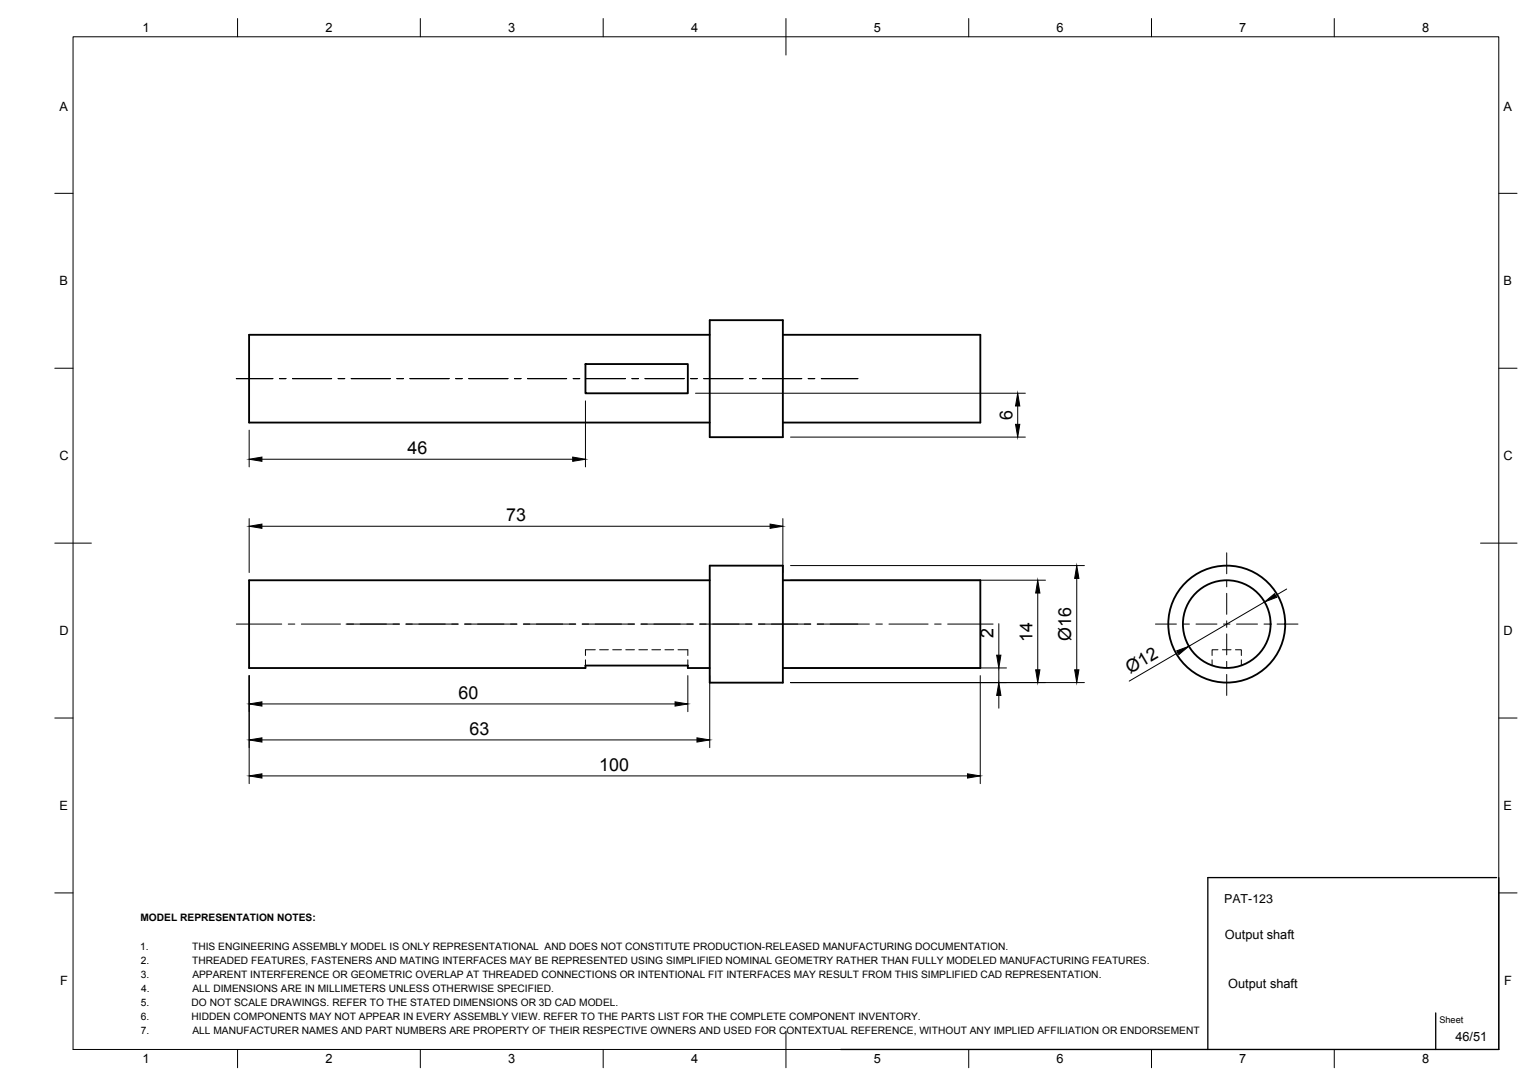
ISO-10303-21;
HEADER;
/* Generated by software containing ST-Developer
 * from STEP Tools, Inc. (www.steptools.com) 
 */

FILE_DESCRIPTION(
/* description */ ('Worm-less right-angle friction wheel drive'),
/* implementation_level */ '2;1');

FILE_NAME(
/* name */ 'Output shaft.step',
/* time_stamp */ '2026-10-28T03:22:36-07:00',
/* author */ (''),
/* organization */ (''),
/* preprocessor_version */ 'ST-DEVELOPER v20.2',
/* originating_system */ 'Autodesk Translation Framework v15.17.0.0',
/* authorisation */ '');

FILE_SCHEMA (('AUTOMOTIVE_DESIGN { 1 0 10303 214 3 1 1 }'));
ENDSEC;

DATA;
#10=MECHANICAL_DESIGN_GEOMETRIC_PRESENTATION_REPRESENTATION('',(#657),#17046);
#556=SHAPE_REPRESENTATION_RELATIONSHIP('SRR','None',#17302,#603);
#603=ADVANCED_BREP_SHAPE_REPRESENTATION('',(#707),#17038);
#657=STYLED_ITEM('',(#17591),#707);
#707=MANIFOLD_SOLID_BREP('Body1',#8216);
#937=FACE_BOUND('',#2304,.T.);
#938=FACE_BOUND('',#2306,.T.);
#939=FACE_BOUND('',#2310,.T.);
#1162=PLANE('',#9644);
#1163=PLANE('',#9645);
#1164=PLANE('',#9647);
#1165=PLANE('',#9648);
#1166=PLANE('',#9649);
#1167=PLANE('',#9651);
#1168=PLANE('',#9654);
#1169=PLANE('',#9662);
#1170=PLANE('',#9663);
#1610=FACE_OUTER_BOUND('',#2298,.T.);
#1611=FACE_OUTER_BOUND('',#2299,.T.);
#1612=FACE_OUTER_BOUND('',#2300,.T.);
#1613=FACE_OUTER_BOUND('',#2301,.T.);
#1614=FACE_OUTER_BOUND('',#2302,.T.);
#1615=FACE_OUTER_BOUND('',#2303,.T.);
#1616=FACE_OUTER_BOUND('',#2305,.T.);
#1617=FACE_OUTER_BOUND('',#2307,.T.);
#1618=FACE_OUTER_BOUND('',#2308,.T.);
#1619=FACE_OUTER_BOUND('',#2309,.T.);
#1620=FACE_OUTER_BOUND('',#2311,.T.);
#1621=FACE_OUTER_BOUND('',#2312,.T.);
#2298=EDGE_LOOP('',(#7254,#7255,#7256,#7257));
#2299=EDGE_LOOP('',(#7258,#7259,#7260,#7261));
#2300=EDGE_LOOP('',(#7262,#7263,#7264,#7265));
#2301=EDGE_LOOP('',(#7266,#7267,#7268,#7269));
#2302=EDGE_LOOP('',(#7270,#7271,#7272,#7273));
#2303=EDGE_LOOP('',(#7274));
#2304=EDGE_LOOP('',(#7275));
#2305=EDGE_LOOP('',(#7276));
#2306=EDGE_LOOP('',(#7277));
#2307=EDGE_LOOP('',(#7278,#7279,#7280,#7281));
#2308=EDGE_LOOP('',(#7282,#7283,#7284,#7285));
#2309=EDGE_LOOP('',(#7286,#7287,#7288,#7289));
#2310=EDGE_LOOP('',(#7290,#7291,#7292,#7293));
#2311=EDGE_LOOP('',(#7294));
#2312=EDGE_LOOP('',(#7295));
#2830=LINE('',#16513,#3370);
#2831=LINE('',#16515,#3371);
#2832=LINE('',#16517,#3372);
#2833=LINE('',#16518,#3373);
#2834=LINE('',#16523,#3374);
#2835=LINE('',#16524,#3375);
#2836=LINE('',#16527,#3376);
#2837=LINE('',#16528,#3377);
#2838=LINE('',#16531,#3378);
#2839=LINE('',#16532,#3379);
#2840=LINE('',#16546,#3380);
#2841=LINE('',#16549,#3381);
#2842=LINE('',#16554,#3382);
#3370=VECTOR('',#12032,1.);
#3371=VECTOR('',#12033,1.);
#3372=VECTOR('',#12034,1.);
#3373=VECTOR('',#12035,1.);
#3374=VECTOR('',#12040,1.);
#3375=VECTOR('',#12041,1.);
#3376=VECTOR('',#12044,1.);
#3377=VECTOR('',#12045,1.);
#3378=VECTOR('',#12048,1.);
#3379=VECTOR('',#12049,1.);
#3380=VECTOR('',#12068,0.8);
#3381=VECTOR('',#12071,0.6);
#3382=VECTOR('',#12078,0.6);
#3832=CIRCLE('',#9646,0.6);
#3833=CIRCLE('',#9650,0.6);
#3834=CIRCLE('',#9652,0.8);
#3835=CIRCLE('',#9653,0.6);
#3836=CIRCLE('',#9655,0.8);
#3837=CIRCLE('',#9656,0.6);
#3838=CIRCLE('',#9659,0.6);
#3839=CIRCLE('',#9661,0.6);
#4445=VERTEX_POINT('',#16511);
#4446=VERTEX_POINT('',#16512);
#4447=VERTEX_POINT('',#16514);
#4448=VERTEX_POINT('',#16516);
#4449=VERTEX_POINT('',#16520);
#4450=VERTEX_POINT('',#16522);
#4451=VERTEX_POINT('',#16526);
#4452=VERTEX_POINT('',#16530);
#4453=VERTEX_POINT('',#16536);
#4454=VERTEX_POINT('',#16538);
#4455=VERTEX_POINT('',#16541);
#4456=VERTEX_POINT('',#16543);
#4457=VERTEX_POINT('',#16548);
#4458=VERTEX_POINT('',#16552);
#5396=EDGE_CURVE('',#4445,#4446,#2830,.T.);
#5397=EDGE_CURVE('',#4445,#4447,#2831,.T.);
#5398=EDGE_CURVE('',#4448,#4447,#2832,.T.);
#5399=EDGE_CURVE('',#4446,#4448,#2833,.T.);
#5400=EDGE_CURVE('',#4446,#4449,#3832,.T.);
#5401=EDGE_CURVE('',#4448,#4450,#2834,.T.);
#5402=EDGE_CURVE('',#4450,#4449,#2835,.T.);
#5403=EDGE_CURVE('',#4447,#4451,#2836,.T.);
#5404=EDGE_CURVE('',#4450,#4451,#2837,.T.);
#5405=EDGE_CURVE('',#4449,#4452,#2838,.T.);
#5406=EDGE_CURVE('',#4451,#4452,#2839,.T.);
#5407=EDGE_CURVE('',#4452,#4445,#3833,.T.);
#5408=EDGE_CURVE('',#4453,#4453,#3834,.T.);
#5409=EDGE_CURVE('',#4454,#4454,#3835,.T.);
#5410=EDGE_CURVE('',#4455,#4455,#3836,.T.);
#5411=EDGE_CURVE('',#4456,#4456,#3837,.T.);
#5412=EDGE_CURVE('',#4453,#4455,#2840,.T.);
#5413=EDGE_CURVE('',#4456,#4457,#2841,.T.);
#5414=EDGE_CURVE('',#4457,#4457,#3838,.T.);
#5415=EDGE_CURVE('',#4458,#4458,#3839,.T.);
#5416=EDGE_CURVE('',#4458,#4454,#2842,.T.);
#7254=ORIENTED_EDGE('',*,*,#5396,.F.);
#7255=ORIENTED_EDGE('',*,*,#5397,.T.);
#7256=ORIENTED_EDGE('',*,*,#5398,.F.);
#7257=ORIENTED_EDGE('',*,*,#5399,.F.);
#7258=ORIENTED_EDGE('',*,*,#5400,.F.);
#7259=ORIENTED_EDGE('',*,*,#5399,.T.);
#7260=ORIENTED_EDGE('',*,*,#5401,.T.);
#7261=ORIENTED_EDGE('',*,*,#5402,.T.);
#7262=ORIENTED_EDGE('',*,*,#5401,.F.);
#7263=ORIENTED_EDGE('',*,*,#5398,.T.);
#7264=ORIENTED_EDGE('',*,*,#5403,.T.);
#7265=ORIENTED_EDGE('',*,*,#5404,.F.);
#7266=ORIENTED_EDGE('',*,*,#5405,.F.);
#7267=ORIENTED_EDGE('',*,*,#5402,.F.);
#7268=ORIENTED_EDGE('',*,*,#5404,.T.);
#7269=ORIENTED_EDGE('',*,*,#5406,.T.);
#7270=ORIENTED_EDGE('',*,*,#5407,.F.);
#7271=ORIENTED_EDGE('',*,*,#5406,.F.);
#7272=ORIENTED_EDGE('',*,*,#5403,.F.);
#7273=ORIENTED_EDGE('',*,*,#5397,.F.);
#7274=ORIENTED_EDGE('',*,*,#5408,.T.);
#7275=ORIENTED_EDGE('',*,*,#5409,.F.);
#7276=ORIENTED_EDGE('',*,*,#5410,.F.);
#7277=ORIENTED_EDGE('',*,*,#5411,.F.);
#7278=ORIENTED_EDGE('',*,*,#5408,.F.);
#7279=ORIENTED_EDGE('',*,*,#5412,.T.);
#7280=ORIENTED_EDGE('',*,*,#5410,.T.);
#7281=ORIENTED_EDGE('',*,*,#5412,.F.);
#7282=ORIENTED_EDGE('',*,*,#5411,.T.);
#7283=ORIENTED_EDGE('',*,*,#5413,.T.);
#7284=ORIENTED_EDGE('',*,*,#5414,.T.);
#7285=ORIENTED_EDGE('',*,*,#5413,.F.);
#7286=ORIENTED_EDGE('',*,*,#5415,.F.);
#7287=ORIENTED_EDGE('',*,*,#5416,.T.);
#7288=ORIENTED_EDGE('',*,*,#5409,.T.);
#7289=ORIENTED_EDGE('',*,*,#5416,.F.);
#7290=ORIENTED_EDGE('',*,*,#5405,.T.);
#7291=ORIENTED_EDGE('',*,*,#5407,.T.);
#7292=ORIENTED_EDGE('',*,*,#5396,.T.);
#7293=ORIENTED_EDGE('',*,*,#5400,.T.);
#7294=ORIENTED_EDGE('',*,*,#5415,.T.);
#7295=ORIENTED_EDGE('',*,*,#5414,.F.);
#7683=CYLINDRICAL_SURFACE('',#9657,0.8);
#7684=CYLINDRICAL_SURFACE('',#9658,0.6);
#7685=CYLINDRICAL_SURFACE('',#9660,0.6);
#8102=ADVANCED_FACE('',(#1610),#1162,.F.);
#8103=ADVANCED_FACE('',(#1611),#1163,.T.);
#8104=ADVANCED_FACE('',(#1612),#1164,.F.);
#8105=ADVANCED_FACE('',(#1613),#1165,.F.);
#8106=ADVANCED_FACE('',(#1614),#1166,.F.);
#8107=ADVANCED_FACE('',(#1615,#937),#1167,.T.);
#8108=ADVANCED_FACE('',(#1616,#938),#1168,.F.);
#8109=ADVANCED_FACE('',(#1617),#7683,.T.);
#8110=ADVANCED_FACE('',(#1618),#7684,.T.);
#8111=ADVANCED_FACE('',(#1619,#939),#7685,.T.);
#8112=ADVANCED_FACE('',(#1620),#1169,.T.);
#8113=ADVANCED_FACE('',(#1621),#1170,.F.);
#8216=CLOSED_SHELL('',(#8102,#8103,#8104,#8105,#8106,#8107,#8108,#8109,
#8110,#8111,#8112,#8113));
#9643=AXIS2_PLACEMENT_3D('',#16509,#12028,#12029);
#9644=AXIS2_PLACEMENT_3D('',#16510,#12030,#12031);
#9645=AXIS2_PLACEMENT_3D('',#16519,#12036,#12037);
#9646=AXIS2_PLACEMENT_3D('',#16521,#12038,#12039);
#9647=AXIS2_PLACEMENT_3D('',#16525,#12042,#12043);
#9648=AXIS2_PLACEMENT_3D('',#16529,#12046,#12047);
#9649=AXIS2_PLACEMENT_3D('',#16533,#12050,#12051);
#9650=AXIS2_PLACEMENT_3D('',#16534,#12052,#12053);
#9651=AXIS2_PLACEMENT_3D('',#16535,#12054,#12055);
#9652=AXIS2_PLACEMENT_3D('',#16537,#12056,#12057);
#9653=AXIS2_PLACEMENT_3D('',#16539,#12058,#12059);
#9654=AXIS2_PLACEMENT_3D('',#16540,#12060,#12061);
#9655=AXIS2_PLACEMENT_3D('',#16542,#12062,#12063);
#9656=AXIS2_PLACEMENT_3D('',#16544,#12064,#12065);
#9657=AXIS2_PLACEMENT_3D('',#16545,#12066,#12067);
#9658=AXIS2_PLACEMENT_3D('',#16547,#12069,#12070);
#9659=AXIS2_PLACEMENT_3D('',#16550,#12072,#12073);
#9660=AXIS2_PLACEMENT_3D('',#16551,#12074,#12075);
#9661=AXIS2_PLACEMENT_3D('',#16553,#12076,#12077);
#9662=AXIS2_PLACEMENT_3D('',#16555,#12079,#12080);
#9663=AXIS2_PLACEMENT_3D('',#16556,#12081,#12082);
#12028=DIRECTION('axis',(0.,0.,1.));
#12029=DIRECTION('refdir',(1.,0.,0.));
#12030=DIRECTION('center_axis',(0.,1.,0.));
#12031=DIRECTION('ref_axis',(0.,0.,1.));
#12032=DIRECTION('',(-1.,0.,0.));
#12033=DIRECTION('',(0.,0.,1.));
#12034=DIRECTION('',(1.,0.,0.));
#12035=DIRECTION('',(0.,0.,1.));
#12036=DIRECTION('center_axis',(1.,0.,0.));
#12037=DIRECTION('ref_axis',(0.,0.,-1.));
#12038=DIRECTION('center_axis',(-1.,0.,0.));
#12039=DIRECTION('ref_axis',(0.,0.,-1.));
#12040=DIRECTION('',(0.,-1.,0.));
#12041=DIRECTION('',(0.,0.,-1.));
#12042=DIRECTION('center_axis',(0.,0.,1.));
#12043=DIRECTION('ref_axis',(0.,-1.,0.));
#12044=DIRECTION('',(0.,-1.,0.));
#12045=DIRECTION('',(1.,0.,0.));
#12046=DIRECTION('center_axis',(0.,-1.,0.));
#12047=DIRECTION('ref_axis',(0.,0.,-1.));
#12048=DIRECTION('',(1.,0.,0.));
#12049=DIRECTION('',(0.,0.,-1.));
#12050=DIRECTION('center_axis',(1.,0.,0.));
#12051=DIRECTION('ref_axis',(0.,0.,-1.));
#12052=DIRECTION('center_axis',(1.,0.,0.));
#12053=DIRECTION('ref_axis',(0.,0.,-1.));
#12054=DIRECTION('center_axis',(1.,0.,0.));
#12055=DIRECTION('ref_axis',(0.,0.,-1.));
#12056=DIRECTION('center_axis',(1.,0.,0.));
#12057=DIRECTION('ref_axis',(0.,0.,-1.));
#12058=DIRECTION('center_axis',(1.,0.,0.));
#12059=DIRECTION('ref_axis',(0.,0.,-1.));
#12060=DIRECTION('center_axis',(1.,0.,0.));
#12061=DIRECTION('ref_axis',(0.,0.,-1.));
#12062=DIRECTION('center_axis',(1.,0.,0.));
#12063=DIRECTION('ref_axis',(0.,0.,-1.));
#12064=DIRECTION('center_axis',(-1.,0.,0.));
#12065=DIRECTION('ref_axis',(0.,0.,-1.));
#12066=DIRECTION('center_axis',(1.,0.,0.));
#12067=DIRECTION('ref_axis',(0.,0.,-1.));
#12068=DIRECTION('',(-1.,0.,0.));
#12069=DIRECTION('center_axis',(1.,0.,0.));
#12070=DIRECTION('ref_axis',(0.,0.,-1.));
#12071=DIRECTION('',(-1.,0.,0.));
#12072=DIRECTION('center_axis',(1.,0.,0.));
#12073=DIRECTION('ref_axis',(0.,0.,-1.));
#12074=DIRECTION('center_axis',(1.,0.,0.));
#12075=DIRECTION('ref_axis',(0.,0.,-1.));
#12076=DIRECTION('center_axis',(1.,0.,0.));
#12077=DIRECTION('ref_axis',(0.,0.,-1.));
#12078=DIRECTION('',(-1.,0.,0.));
#12079=DIRECTION('center_axis',(1.,0.,0.));
#12080=DIRECTION('ref_axis',(0.,0.,-1.));
#12081=DIRECTION('center_axis',(1.,0.,0.));
#12082=DIRECTION('ref_axis',(0.,0.,-1.));
#16509=CARTESIAN_POINT('',(0.,0.,0.));
#16510=CARTESIAN_POINT('Origin',(1.5,3.2,6.3));
#16511=CARTESIAN_POINT('',(2.9,3.2,6.43431457505076));
#16512=CARTESIAN_POINT('',(1.5,3.2,6.43431457505076));
#16513=CARTESIAN_POINT('',(-2.5,3.2,6.43431457505076));
#16514=CARTESIAN_POINT('',(2.9,3.2,6.65));
#16515=CARTESIAN_POINT('',(2.9,3.2,6.3));
#16516=CARTESIAN_POINT('',(1.5,3.2,6.65));
#16517=CARTESIAN_POINT('',(1.5,3.2,6.65));
#16518=CARTESIAN_POINT('',(1.5,3.2,6.3));
#16519=CARTESIAN_POINT('Origin',(1.5,3.,6.475));
#16520=CARTESIAN_POINT('',(1.5,2.8,6.43431457505076));
#16521=CARTESIAN_POINT('Origin',(1.5,3.,7.));
#16522=CARTESIAN_POINT('',(1.5,2.8,6.65));
#16523=CARTESIAN_POINT('',(1.5,3.2,6.65));
#16524=CARTESIAN_POINT('',(1.5,2.8,6.65));
#16525=CARTESIAN_POINT('Origin',(1.5,3.2,6.65));
#16526=CARTESIAN_POINT('',(2.9,2.8,6.65));
#16527=CARTESIAN_POINT('',(2.9,3.2,6.65));
#16528=CARTESIAN_POINT('',(1.5,2.8,6.65));
#16529=CARTESIAN_POINT('Origin',(1.5,2.8,6.65));
#16530=CARTESIAN_POINT('',(2.9,2.8,6.43431457505076));
#16531=CARTESIAN_POINT('',(-2.5,2.8,6.43431457505076));
#16532=CARTESIAN_POINT('',(2.9,2.8,6.65));
#16533=CARTESIAN_POINT('Origin',(2.9,3.,6.475));
#16534=CARTESIAN_POINT('Origin',(2.9,3.,7.));
#16535=CARTESIAN_POINT('Origin',(1.2,3.,7.));
#16536=CARTESIAN_POINT('',(1.2,3.,7.8));
#16537=CARTESIAN_POINT('Origin',(1.2,3.,7.));
#16538=CARTESIAN_POINT('',(1.2,3.,7.6));
#16539=CARTESIAN_POINT('Origin',(1.2,3.,7.));
#16540=CARTESIAN_POINT('Origin',(0.2,3.,7.));
#16541=CARTESIAN_POINT('',(0.2,3.,7.8));
#16542=CARTESIAN_POINT('Origin',(0.2,3.,7.));
#16543=CARTESIAN_POINT('',(0.2,3.,7.6));
#16544=CARTESIAN_POINT('Origin',(0.2,3.,7.));
#16545=CARTESIAN_POINT('Origin',(0.2,3.,7.));
#16546=CARTESIAN_POINT('',(0.2,3.,7.8));
#16547=CARTESIAN_POINT('Origin',(-2.5,3.,7.));
#16548=CARTESIAN_POINT('',(-2.5,3.,7.6));
#16549=CARTESIAN_POINT('',(-2.5,3.,7.6));
#16550=CARTESIAN_POINT('Origin',(-2.5,3.,7.));
#16551=CARTESIAN_POINT('Origin',(-2.5,3.,7.));
#16552=CARTESIAN_POINT('',(7.5,3.,7.6));
#16553=CARTESIAN_POINT('Origin',(7.5,3.,7.));
#16554=CARTESIAN_POINT('',(-2.5,3.,7.6));
#16555=CARTESIAN_POINT('Origin',(7.5,3.,7.));
#16556=CARTESIAN_POINT('Origin',(-2.5,3.,7.));
#16985=UNCERTAINTY_MEASURE_WITH_UNIT(LENGTH_MEASURE(0.001),#17047,
'DISTANCE_ACCURACY_VALUE',
'Maximum model space distance between geometric entities at asserted c
onnectivities');
#16993=UNCERTAINTY_MEASURE_WITH_UNIT(LENGTH_MEASURE(0.001),#17047,
'DISTANCE_ACCURACY_VALUE',
'Maximum model space distance between geometric entities at asserted c
onnectivities');
#17038=(
GEOMETRIC_REPRESENTATION_CONTEXT(3)
GLOBAL_UNCERTAINTY_ASSIGNED_CONTEXT((#16985))
GLOBAL_UNIT_ASSIGNED_CONTEXT((#17047,#17049,#17050))
REPRESENTATION_CONTEXT('','3D')
);
#17046=(
GEOMETRIC_REPRESENTATION_CONTEXT(3)
GLOBAL_UNCERTAINTY_ASSIGNED_CONTEXT((#16993))
GLOBAL_UNIT_ASSIGNED_CONTEXT((#17047,#17049,#17050))
REPRESENTATION_CONTEXT('','3D')
);
#17047=(
LENGTH_UNIT()
NAMED_UNIT(*)
SI_UNIT(.CENTI.,.METRE.)
);
#17049=(
NAMED_UNIT(*)
PLANE_ANGLE_UNIT()
SI_UNIT($,.RADIAN.)
);
#17050=(
NAMED_UNIT(*)
SI_UNIT($,.STERADIAN.)
SOLID_ANGLE_UNIT()
);
#17095=SHAPE_DEFINITION_REPRESENTATION(#17229,#17302);
#17229=PRODUCT_DEFINITION_SHAPE('',$,#17355);
#17302=SHAPE_REPRESENTATION('',(#9643),#17038);
#17310=PRODUCT_DEFINITION_CONTEXT('part definition',#17468,'design');
#17355=PRODUCT_DEFINITION('Output shaft','Output shaft',#17407,#17310);
#17407=PRODUCT_DEFINITION_FORMATION('',$,#17514);
#17468=APPLICATION_CONTEXT(
'Core Data for Automotive Mechanical Design Process');
#17469=PRODUCT_CONTEXT('part definition',#17468,'mechanical');
#17514=PRODUCT('Output shaft','Output shaft','Output shaft',(#17469));
#17585=COLOUR_RGB('Grey',0.48,0.52,0.57);
#17586=FILL_AREA_STYLE_COLOUR('',#17585);
#17587=FILL_AREA_STYLE('',(#17586));
#17588=SURFACE_STYLE_FILL_AREA(#17587);
#17589=SURFACE_SIDE_STYLE('',(#17588));
#17590=SURFACE_STYLE_USAGE(.BOTH.,#17589);
#17591=PRESENTATION_STYLE_ASSIGNMENT((#17590));
ENDSEC;
END-ISO-10303-21;
